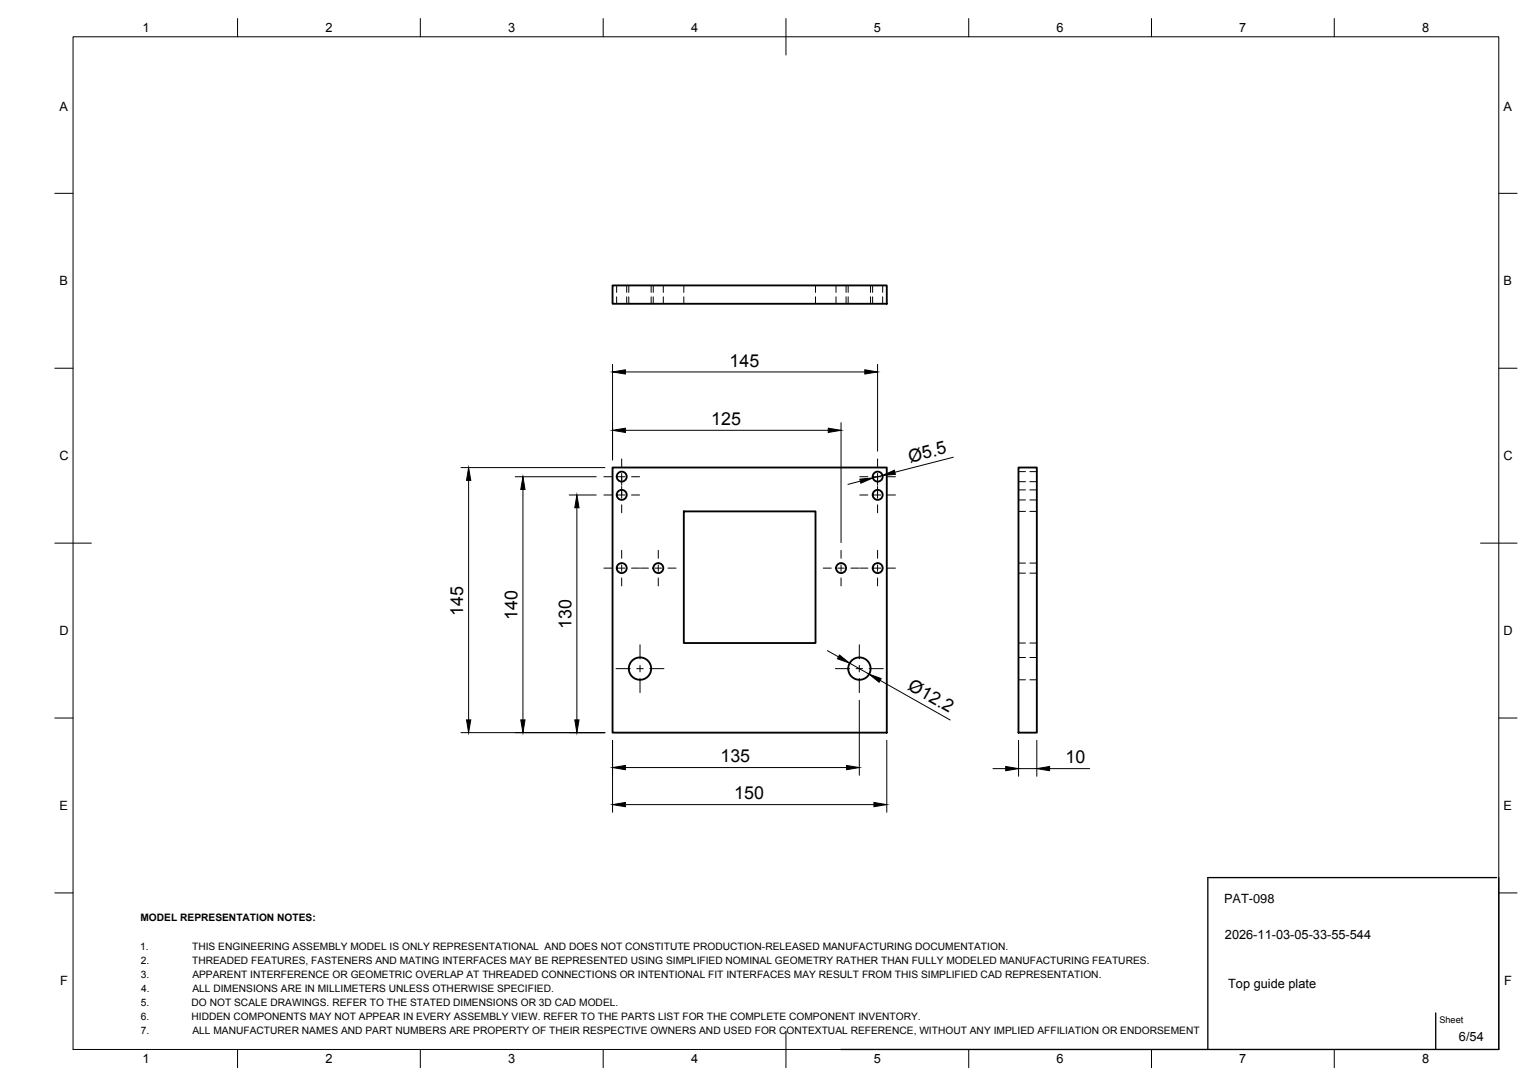
ISO-10303-21;
HEADER;
/* Generated by software containing ST-Developer
 * from STEP Tools, Inc. (www.steptools.com) 
 */

FILE_DESCRIPTION(
/* description */ ('Spring compression tester'),
/* implementation_level */ '2;1');

FILE_NAME(
/* name */ 'Top guide plate.step',
/* time_stamp */ '2026-10-28T03:24:11-07:00',
/* author */ (''),
/* organization */ (''),
/* preprocessor_version */ 'ST-DEVELOPER v20.2',
/* originating_system */ 'Autodesk Translation Framework v15.17.0.0',
/* authorisation */ '');

FILE_SCHEMA (('AUTOMOTIVE_DESIGN { 1 0 10303 214 3 1 1 }'));
ENDSEC;

DATA;
#10=MECHANICAL_DESIGN_GEOMETRIC_PRESENTATION_REPRESENTATION('',(#1107),#43521);
#987=SHAPE_REPRESENTATION_RELATIONSHIP('SRR','None',#43799,#1047);
#1047=ADVANCED_BREP_SHAPE_REPRESENTATION('',(#1182),#43459);
#1107=STYLED_ITEM('',(#44195),#1182);
#1182=MANIFOLD_SOLID_BREP('Body1',#18544);
#1283=FACE_BOUND('',#3318,.T.);
#1284=FACE_BOUND('',#3319,.T.);
#1285=FACE_BOUND('',#3320,.T.);
#1286=FACE_BOUND('',#3321,.T.);
#1287=FACE_BOUND('',#3322,.T.);
#1288=FACE_BOUND('',#3323,.T.);
#1289=FACE_BOUND('',#3324,.T.);
#1290=FACE_BOUND('',#3325,.T.);
#1291=FACE_BOUND('',#3326,.T.);
#1292=FACE_BOUND('',#3327,.T.);
#1293=FACE_BOUND('',#3328,.T.);
#1294=FACE_BOUND('',#3330,.T.);
#1295=FACE_BOUND('',#3331,.T.);
#1296=FACE_BOUND('',#3332,.T.);
#1297=FACE_BOUND('',#3333,.T.);
#1298=FACE_BOUND('',#3334,.T.);
#1299=FACE_BOUND('',#3335,.T.);
#1300=FACE_BOUND('',#3336,.T.);
#1301=FACE_BOUND('',#3337,.T.);
#1302=FACE_BOUND('',#3338,.T.);
#1303=FACE_BOUND('',#3339,.T.);
#1304=FACE_BOUND('',#3340,.T.);
#1615=PLANE('',#19400);
#1616=PLANE('',#19401);
#1617=PLANE('',#19402);
#1618=PLANE('',#19403);
#1619=PLANE('',#19410);
#1620=PLANE('',#19411);
#1621=PLANE('',#19412);
#1622=PLANE('',#19413);
#1623=PLANE('',#19414);
#1624=PLANE('',#19415);
#2216=FACE_OUTER_BOUND('',#3299,.T.);
#2217=FACE_OUTER_BOUND('',#3300,.T.);
#2218=FACE_OUTER_BOUND('',#3301,.T.);
#2219=FACE_OUTER_BOUND('',#3302,.T.);
#2220=FACE_OUTER_BOUND('',#3303,.T.);
#2221=FACE_OUTER_BOUND('',#3304,.T.);
#2222=FACE_OUTER_BOUND('',#3305,.T.);
#2223=FACE_OUTER_BOUND('',#3306,.T.);
#2224=FACE_OUTER_BOUND('',#3307,.T.);
#2225=FACE_OUTER_BOUND('',#3308,.T.);
#2226=FACE_OUTER_BOUND('',#3309,.T.);
#2227=FACE_OUTER_BOUND('',#3310,.T.);
#2228=FACE_OUTER_BOUND('',#3311,.T.);
#2229=FACE_OUTER_BOUND('',#3312,.T.);
#2230=FACE_OUTER_BOUND('',#3313,.T.);
#2231=FACE_OUTER_BOUND('',#3314,.T.);
#2232=FACE_OUTER_BOUND('',#3315,.T.);
#2233=FACE_OUTER_BOUND('',#3316,.T.);
#2234=FACE_OUTER_BOUND('',#3317,.T.);
#2235=FACE_OUTER_BOUND('',#3329,.T.);
#3299=EDGE_LOOP('',(#12433,#12434,#12435,#12436));
#3300=EDGE_LOOP('',(#12437,#12438,#12439,#12440));
#3301=EDGE_LOOP('',(#12441,#12442,#12443,#12444));
#3302=EDGE_LOOP('',(#12445,#12446,#12447,#12448));
#3303=EDGE_LOOP('',(#12449,#12450,#12451,#12452));
#3304=EDGE_LOOP('',(#12453,#12454,#12455,#12456));
#3305=EDGE_LOOP('',(#12457,#12458,#12459,#12460));
#3306=EDGE_LOOP('',(#12461,#12462,#12463,#12464));
#3307=EDGE_LOOP('',(#12465,#12466,#12467,#12468));
#3308=EDGE_LOOP('',(#12469,#12470,#12471,#12472));
#3309=EDGE_LOOP('',(#12473,#12474,#12475,#12476));
#3310=EDGE_LOOP('',(#12477,#12478,#12479,#12480));
#3311=EDGE_LOOP('',(#12481,#12482,#12483,#12484));
#3312=EDGE_LOOP('',(#12485,#12486,#12487,#12488));
#3313=EDGE_LOOP('',(#12489,#12490,#12491,#12492));
#3314=EDGE_LOOP('',(#12493,#12494,#12495,#12496));
#3315=EDGE_LOOP('',(#12497,#12498,#12499,#12500));
#3316=EDGE_LOOP('',(#12501,#12502,#12503,#12504));
#3317=EDGE_LOOP('',(#12505,#12506,#12507,#12508));
#3318=EDGE_LOOP('',(#12509));
#3319=EDGE_LOOP('',(#12510));
#3320=EDGE_LOOP('',(#12511));
#3321=EDGE_LOOP('',(#12512));
#3322=EDGE_LOOP('',(#12513,#12514,#12515,#12516));
#3323=EDGE_LOOP('',(#12517));
#3324=EDGE_LOOP('',(#12518));
#3325=EDGE_LOOP('',(#12519));
#3326=EDGE_LOOP('',(#12520));
#3327=EDGE_LOOP('',(#12521));
#3328=EDGE_LOOP('',(#12522));
#3329=EDGE_LOOP('',(#12523,#12524,#12525,#12526));
#3330=EDGE_LOOP('',(#12527));
#3331=EDGE_LOOP('',(#12528));
#3332=EDGE_LOOP('',(#12529));
#3333=EDGE_LOOP('',(#12530));
#3334=EDGE_LOOP('',(#12531,#12532,#12533,#12534));
#3335=EDGE_LOOP('',(#12535));
#3336=EDGE_LOOP('',(#12536));
#3337=EDGE_LOOP('',(#12537));
#3338=EDGE_LOOP('',(#12538));
#3339=EDGE_LOOP('',(#12539));
#3340=EDGE_LOOP('',(#12540));
#4674=LINE('',#26688,#6106);
#4675=LINE('',#26694,#6107);
#4676=LINE('',#26700,#6108);
#4677=LINE('',#26706,#6109);
#4678=LINE('',#26712,#6110);
#4679=LINE('',#26718,#6111);
#4680=LINE('',#26724,#6112);
#4681=LINE('',#26730,#6113);
#4682=LINE('',#26735,#6114);
#4683=LINE('',#26737,#6115);
#4684=LINE('',#26739,#6116);
#4685=LINE('',#26740,#6117);
#4686=LINE('',#26743,#6118);
#4687=LINE('',#26745,#6119);
#4688=LINE('',#26746,#6120);
#4689=LINE('',#26749,#6121);
#4690=LINE('',#26751,#6122);
#4691=LINE('',#26752,#6123);
#4692=LINE('',#26754,#6124);
#4693=LINE('',#26755,#6125);
#4694=LINE('',#26760,#6126);
#4695=LINE('',#26766,#6127);
#4696=LINE('',#26771,#6128);
#4697=LINE('',#26773,#6129);
#4698=LINE('',#26775,#6130);
#4699=LINE('',#26776,#6131);
#4700=LINE('',#26779,#6132);
#4701=LINE('',#26781,#6133);
#4702=LINE('',#26782,#6134);
#4703=LINE('',#26785,#6135);
#4704=LINE('',#26787,#6136);
#4705=LINE('',#26788,#6137);
#4706=LINE('',#26790,#6138);
#4707=LINE('',#26791,#6139);
#6106=VECTOR('',#21452,0.275);
#6107=VECTOR('',#21459,0.275);
#6108=VECTOR('',#21466,0.275);
#6109=VECTOR('',#21473,0.275);
#6110=VECTOR('',#21480,0.275);
#6111=VECTOR('',#21487,0.275);
#6112=VECTOR('',#21494,0.275);
#6113=VECTOR('',#21501,0.275);
#6114=VECTOR('',#21506,1.);
#6115=VECTOR('',#21507,1.);
#6116=VECTOR('',#21508,1.);
#6117=VECTOR('',#21509,1.);
#6118=VECTOR('',#21512,1.);
#6119=VECTOR('',#21513,1.);
#6120=VECTOR('',#21514,1.);
#6121=VECTOR('',#21517,1.);
#6122=VECTOR('',#21518,1.);
#6123=VECTOR('',#21519,1.);
#6124=VECTOR('',#21522,1.);
#6125=VECTOR('',#21523,1.);
#6126=VECTOR('',#21528,0.61);
#6127=VECTOR('',#21535,0.61);
#6128=VECTOR('',#21540,1.);
#6129=VECTOR('',#21541,1.);
#6130=VECTOR('',#21542,1.);
#6131=VECTOR('',#21543,1.);
#6132=VECTOR('',#21546,1.);
#6133=VECTOR('',#21547,1.);
#6134=VECTOR('',#21548,1.);
#6135=VECTOR('',#21551,1.);
#6136=VECTOR('',#21552,1.);
#6137=VECTOR('',#21553,1.);
#6138=VECTOR('',#21556,1.);
#6139=VECTOR('',#21557,1.);
#7510=CIRCLE('',#19377,0.275);
#7511=CIRCLE('',#19378,0.275);
#7512=CIRCLE('',#19380,0.275);
#7513=CIRCLE('',#19381,0.275);
#7514=CIRCLE('',#19383,0.275);
#7515=CIRCLE('',#19384,0.275);
#7516=CIRCLE('',#19386,0.275);
#7517=CIRCLE('',#19387,0.275);
#7518=CIRCLE('',#19389,0.275);
#7519=CIRCLE('',#19390,0.275);
#7520=CIRCLE('',#19392,0.275);
#7521=CIRCLE('',#19393,0.275);
#7522=CIRCLE('',#19395,0.275);
#7523=CIRCLE('',#19396,0.275);
#7524=CIRCLE('',#19398,0.275);
#7525=CIRCLE('',#19399,0.275);
#7526=CIRCLE('',#19405,0.61);
#7527=CIRCLE('',#19406,0.61);
#7528=CIRCLE('',#19408,0.61);
#7529=CIRCLE('',#19409,0.61);
#8208=VERTEX_POINT('',#26685);
#8209=VERTEX_POINT('',#26687);
#8210=VERTEX_POINT('',#26691);
#8211=VERTEX_POINT('',#26693);
#8212=VERTEX_POINT('',#26697);
#8213=VERTEX_POINT('',#26699);
#8214=VERTEX_POINT('',#26703);
#8215=VERTEX_POINT('',#26705);
#8216=VERTEX_POINT('',#26709);
#8217=VERTEX_POINT('',#26711);
#8218=VERTEX_POINT('',#26715);
#8219=VERTEX_POINT('',#26717);
#8220=VERTEX_POINT('',#26721);
#8221=VERTEX_POINT('',#26723);
#8222=VERTEX_POINT('',#26727);
#8223=VERTEX_POINT('',#26729);
#8224=VERTEX_POINT('',#26733);
#8225=VERTEX_POINT('',#26734);
#8226=VERTEX_POINT('',#26736);
#8227=VERTEX_POINT('',#26738);
#8228=VERTEX_POINT('',#26742);
#8229=VERTEX_POINT('',#26744);
#8230=VERTEX_POINT('',#26748);
#8231=VERTEX_POINT('',#26750);
#8232=VERTEX_POINT('',#26757);
#8233=VERTEX_POINT('',#26759);
#8234=VERTEX_POINT('',#26763);
#8235=VERTEX_POINT('',#26765);
#8236=VERTEX_POINT('',#26769);
#8237=VERTEX_POINT('',#26770);
#8238=VERTEX_POINT('',#26772);
#8239=VERTEX_POINT('',#26774);
#8240=VERTEX_POINT('',#26778);
#8241=VERTEX_POINT('',#26780);
#8242=VERTEX_POINT('',#26784);
#8243=VERTEX_POINT('',#26786);
#9881=EDGE_CURVE('',#8208,#8208,#7510,.T.);
#9882=EDGE_CURVE('',#8208,#8209,#4674,.T.);
#9883=EDGE_CURVE('',#8209,#8209,#7511,.T.);
#9884=EDGE_CURVE('',#8210,#8210,#7512,.T.);
#9885=EDGE_CURVE('',#8210,#8211,#4675,.T.);
#9886=EDGE_CURVE('',#8211,#8211,#7513,.T.);
#9887=EDGE_CURVE('',#8212,#8212,#7514,.T.);
#9888=EDGE_CURVE('',#8212,#8213,#4676,.T.);
#9889=EDGE_CURVE('',#8213,#8213,#7515,.T.);
#9890=EDGE_CURVE('',#8214,#8214,#7516,.T.);
#9891=EDGE_CURVE('',#8214,#8215,#4677,.T.);
#9892=EDGE_CURVE('',#8215,#8215,#7517,.T.);
#9893=EDGE_CURVE('',#8216,#8216,#7518,.T.);
#9894=EDGE_CURVE('',#8216,#8217,#4678,.T.);
#9895=EDGE_CURVE('',#8217,#8217,#7519,.T.);
#9896=EDGE_CURVE('',#8218,#8218,#7520,.T.);
#9897=EDGE_CURVE('',#8218,#8219,#4679,.T.);
#9898=EDGE_CURVE('',#8219,#8219,#7521,.T.);
#9899=EDGE_CURVE('',#8220,#8220,#7522,.T.);
#9900=EDGE_CURVE('',#8220,#8221,#4680,.T.);
#9901=EDGE_CURVE('',#8221,#8221,#7523,.T.);
#9902=EDGE_CURVE('',#8222,#8222,#7524,.T.);
#9903=EDGE_CURVE('',#8222,#8223,#4681,.T.);
#9904=EDGE_CURVE('',#8223,#8223,#7525,.T.);
#9905=EDGE_CURVE('',#8224,#8225,#4682,.T.);
#9906=EDGE_CURVE('',#8226,#8224,#4683,.T.);
#9907=EDGE_CURVE('',#8227,#8226,#4684,.T.);
#9908=EDGE_CURVE('',#8227,#8225,#4685,.T.);
#9909=EDGE_CURVE('',#8225,#8228,#4686,.T.);
#9910=EDGE_CURVE('',#8229,#8227,#4687,.T.);
#9911=EDGE_CURVE('',#8229,#8228,#4688,.T.);
#9912=EDGE_CURVE('',#8228,#8230,#4689,.T.);
#9913=EDGE_CURVE('',#8231,#8229,#4690,.T.);
#9914=EDGE_CURVE('',#8231,#8230,#4691,.T.);
#9915=EDGE_CURVE('',#8230,#8224,#4692,.T.);
#9916=EDGE_CURVE('',#8226,#8231,#4693,.T.);
#9917=EDGE_CURVE('',#8232,#8232,#7526,.T.);
#9918=EDGE_CURVE('',#8232,#8233,#4694,.T.);
#9919=EDGE_CURVE('',#8233,#8233,#7527,.T.);
#9920=EDGE_CURVE('',#8234,#8234,#7528,.T.);
#9921=EDGE_CURVE('',#8234,#8235,#4695,.T.);
#9922=EDGE_CURVE('',#8235,#8235,#7529,.T.);
#9923=EDGE_CURVE('',#8236,#8237,#4696,.T.);
#9924=EDGE_CURVE('',#8237,#8238,#4697,.T.);
#9925=EDGE_CURVE('',#8239,#8238,#4698,.T.);
#9926=EDGE_CURVE('',#8236,#8239,#4699,.T.);
#9927=EDGE_CURVE('',#8240,#8236,#4700,.T.);
#9928=EDGE_CURVE('',#8241,#8239,#4701,.T.);
#9929=EDGE_CURVE('',#8240,#8241,#4702,.T.);
#9930=EDGE_CURVE('',#8242,#8240,#4703,.T.);
#9931=EDGE_CURVE('',#8243,#8241,#4704,.T.);
#9932=EDGE_CURVE('',#8242,#8243,#4705,.T.);
#9933=EDGE_CURVE('',#8237,#8242,#4706,.T.);
#9934=EDGE_CURVE('',#8238,#8243,#4707,.T.);
#12433=ORIENTED_EDGE('',*,*,#9881,.F.);
#12434=ORIENTED_EDGE('',*,*,#9882,.T.);
#12435=ORIENTED_EDGE('',*,*,#9883,.F.);
#12436=ORIENTED_EDGE('',*,*,#9882,.F.);
#12437=ORIENTED_EDGE('',*,*,#9884,.F.);
#12438=ORIENTED_EDGE('',*,*,#9885,.T.);
#12439=ORIENTED_EDGE('',*,*,#9886,.F.);
#12440=ORIENTED_EDGE('',*,*,#9885,.F.);
#12441=ORIENTED_EDGE('',*,*,#9887,.F.);
#12442=ORIENTED_EDGE('',*,*,#9888,.T.);
#12443=ORIENTED_EDGE('',*,*,#9889,.F.);
#12444=ORIENTED_EDGE('',*,*,#9888,.F.);
#12445=ORIENTED_EDGE('',*,*,#9890,.F.);
#12446=ORIENTED_EDGE('',*,*,#9891,.T.);
#12447=ORIENTED_EDGE('',*,*,#9892,.F.);
#12448=ORIENTED_EDGE('',*,*,#9891,.F.);
#12449=ORIENTED_EDGE('',*,*,#9893,.F.);
#12450=ORIENTED_EDGE('',*,*,#9894,.T.);
#12451=ORIENTED_EDGE('',*,*,#9895,.F.);
#12452=ORIENTED_EDGE('',*,*,#9894,.F.);
#12453=ORIENTED_EDGE('',*,*,#9896,.F.);
#12454=ORIENTED_EDGE('',*,*,#9897,.T.);
#12455=ORIENTED_EDGE('',*,*,#9898,.F.);
#12456=ORIENTED_EDGE('',*,*,#9897,.F.);
#12457=ORIENTED_EDGE('',*,*,#9899,.F.);
#12458=ORIENTED_EDGE('',*,*,#9900,.T.);
#12459=ORIENTED_EDGE('',*,*,#9901,.F.);
#12460=ORIENTED_EDGE('',*,*,#9900,.F.);
#12461=ORIENTED_EDGE('',*,*,#9902,.F.);
#12462=ORIENTED_EDGE('',*,*,#9903,.T.);
#12463=ORIENTED_EDGE('',*,*,#9904,.F.);
#12464=ORIENTED_EDGE('',*,*,#9903,.F.);
#12465=ORIENTED_EDGE('',*,*,#9905,.F.);
#12466=ORIENTED_EDGE('',*,*,#9906,.F.);
#12467=ORIENTED_EDGE('',*,*,#9907,.F.);
#12468=ORIENTED_EDGE('',*,*,#9908,.T.);
#12469=ORIENTED_EDGE('',*,*,#9909,.F.);
#12470=ORIENTED_EDGE('',*,*,#9908,.F.);
#12471=ORIENTED_EDGE('',*,*,#9910,.F.);
#12472=ORIENTED_EDGE('',*,*,#9911,.T.);
#12473=ORIENTED_EDGE('',*,*,#9912,.F.);
#12474=ORIENTED_EDGE('',*,*,#9911,.F.);
#12475=ORIENTED_EDGE('',*,*,#9913,.F.);
#12476=ORIENTED_EDGE('',*,*,#9914,.T.);
#12477=ORIENTED_EDGE('',*,*,#9915,.F.);
#12478=ORIENTED_EDGE('',*,*,#9914,.F.);
#12479=ORIENTED_EDGE('',*,*,#9916,.F.);
#12480=ORIENTED_EDGE('',*,*,#9906,.T.);
#12481=ORIENTED_EDGE('',*,*,#9917,.F.);
#12482=ORIENTED_EDGE('',*,*,#9918,.T.);
#12483=ORIENTED_EDGE('',*,*,#9919,.F.);
#12484=ORIENTED_EDGE('',*,*,#9918,.F.);
#12485=ORIENTED_EDGE('',*,*,#9920,.F.);
#12486=ORIENTED_EDGE('',*,*,#9921,.T.);
#12487=ORIENTED_EDGE('',*,*,#9922,.F.);
#12488=ORIENTED_EDGE('',*,*,#9921,.F.);
#12489=ORIENTED_EDGE('',*,*,#9923,.T.);
#12490=ORIENTED_EDGE('',*,*,#9924,.T.);
#12491=ORIENTED_EDGE('',*,*,#9925,.F.);
#12492=ORIENTED_EDGE('',*,*,#9926,.F.);
#12493=ORIENTED_EDGE('',*,*,#9927,.T.);
#12494=ORIENTED_EDGE('',*,*,#9926,.T.);
#12495=ORIENTED_EDGE('',*,*,#9928,.F.);
#12496=ORIENTED_EDGE('',*,*,#9929,.F.);
#12497=ORIENTED_EDGE('',*,*,#9930,.T.);
#12498=ORIENTED_EDGE('',*,*,#9929,.T.);
#12499=ORIENTED_EDGE('',*,*,#9931,.F.);
#12500=ORIENTED_EDGE('',*,*,#9932,.F.);
#12501=ORIENTED_EDGE('',*,*,#9933,.T.);
#12502=ORIENTED_EDGE('',*,*,#9932,.T.);
#12503=ORIENTED_EDGE('',*,*,#9934,.F.);
#12504=ORIENTED_EDGE('',*,*,#9924,.F.);
#12505=ORIENTED_EDGE('',*,*,#9934,.T.);
#12506=ORIENTED_EDGE('',*,*,#9931,.T.);
#12507=ORIENTED_EDGE('',*,*,#9928,.T.);
#12508=ORIENTED_EDGE('',*,*,#9925,.T.);
#12509=ORIENTED_EDGE('',*,*,#9889,.T.);
#12510=ORIENTED_EDGE('',*,*,#9892,.T.);
#12511=ORIENTED_EDGE('',*,*,#9922,.T.);
#12512=ORIENTED_EDGE('',*,*,#9919,.T.);
#12513=ORIENTED_EDGE('',*,*,#9912,.T.);
#12514=ORIENTED_EDGE('',*,*,#9915,.T.);
#12515=ORIENTED_EDGE('',*,*,#9905,.T.);
#12516=ORIENTED_EDGE('',*,*,#9909,.T.);
#12517=ORIENTED_EDGE('',*,*,#9904,.T.);
#12518=ORIENTED_EDGE('',*,*,#9901,.T.);
#12519=ORIENTED_EDGE('',*,*,#9898,.T.);
#12520=ORIENTED_EDGE('',*,*,#9895,.T.);
#12521=ORIENTED_EDGE('',*,*,#9886,.T.);
#12522=ORIENTED_EDGE('',*,*,#9883,.T.);
#12523=ORIENTED_EDGE('',*,*,#9933,.F.);
#12524=ORIENTED_EDGE('',*,*,#9923,.F.);
#12525=ORIENTED_EDGE('',*,*,#9927,.F.);
#12526=ORIENTED_EDGE('',*,*,#9930,.F.);
#12527=ORIENTED_EDGE('',*,*,#9887,.T.);
#12528=ORIENTED_EDGE('',*,*,#9890,.T.);
#12529=ORIENTED_EDGE('',*,*,#9920,.T.);
#12530=ORIENTED_EDGE('',*,*,#9917,.T.);
#12531=ORIENTED_EDGE('',*,*,#9913,.T.);
#12532=ORIENTED_EDGE('',*,*,#9910,.T.);
#12533=ORIENTED_EDGE('',*,*,#9907,.T.);
#12534=ORIENTED_EDGE('',*,*,#9916,.T.);
#12535=ORIENTED_EDGE('',*,*,#9902,.T.);
#12536=ORIENTED_EDGE('',*,*,#9899,.T.);
#12537=ORIENTED_EDGE('',*,*,#9896,.T.);
#12538=ORIENTED_EDGE('',*,*,#9893,.T.);
#12539=ORIENTED_EDGE('',*,*,#9884,.T.);
#12540=ORIENTED_EDGE('',*,*,#9881,.T.);
#17125=CYLINDRICAL_SURFACE('',#19376,0.275);
#17126=CYLINDRICAL_SURFACE('',#19379,0.275);
#17127=CYLINDRICAL_SURFACE('',#19382,0.275);
#17128=CYLINDRICAL_SURFACE('',#19385,0.275);
#17129=CYLINDRICAL_SURFACE('',#19388,0.275);
#17130=CYLINDRICAL_SURFACE('',#19391,0.275);
#17131=CYLINDRICAL_SURFACE('',#19394,0.275);
#17132=CYLINDRICAL_SURFACE('',#19397,0.275);
#17133=CYLINDRICAL_SURFACE('',#19404,0.61);
#17134=CYLINDRICAL_SURFACE('',#19407,0.61);
#17540=ADVANCED_FACE('',(#2216),#17125,.F.);
#17541=ADVANCED_FACE('',(#2217),#17126,.F.);
#17542=ADVANCED_FACE('',(#2218),#17127,.F.);
#17543=ADVANCED_FACE('',(#2219),#17128,.F.);
#17544=ADVANCED_FACE('',(#2220),#17129,.F.);
#17545=ADVANCED_FACE('',(#2221),#17130,.F.);
#17546=ADVANCED_FACE('',(#2222),#17131,.F.);
#17547=ADVANCED_FACE('',(#2223),#17132,.F.);
#17548=ADVANCED_FACE('',(#2224),#1615,.F.);
#17549=ADVANCED_FACE('',(#2225),#1616,.F.);
#17550=ADVANCED_FACE('',(#2226),#1617,.F.);
#17551=ADVANCED_FACE('',(#2227),#1618,.F.);
#17552=ADVANCED_FACE('',(#2228),#17133,.F.);
#17553=ADVANCED_FACE('',(#2229),#17134,.F.);
#17554=ADVANCED_FACE('',(#2230),#1619,.T.);
#17555=ADVANCED_FACE('',(#2231),#1620,.T.);
#17556=ADVANCED_FACE('',(#2232),#1621,.T.);
#17557=ADVANCED_FACE('',(#2233),#1622,.T.);
#17558=ADVANCED_FACE('',(#2234,#1283,#1284,#1285,#1286,#1287,#1288,#1289,
#1290,#1291,#1292,#1293),#1623,.T.);
#17559=ADVANCED_FACE('',(#2235,#1294,#1295,#1296,#1297,#1298,#1299,#1300,
#1301,#1302,#1303,#1304),#1624,.F.);
#18544=CLOSED_SHELL('',(#17540,#17541,#17542,#17543,#17544,#17545,#17546,
#17547,#17548,#17549,#17550,#17551,#17552,#17553,#17554,#17555,#17556,#17557,
#17558,#17559));
#19375=AXIS2_PLACEMENT_3D('',#26683,#21446,#21447);
#19376=AXIS2_PLACEMENT_3D('',#26684,#21448,#21449);
#19377=AXIS2_PLACEMENT_3D('',#26686,#21450,#21451);
#19378=AXIS2_PLACEMENT_3D('',#26689,#21453,#21454);
#19379=AXIS2_PLACEMENT_3D('',#26690,#21455,#21456);
#19380=AXIS2_PLACEMENT_3D('',#26692,#21457,#21458);
#19381=AXIS2_PLACEMENT_3D('',#26695,#21460,#21461);
#19382=AXIS2_PLACEMENT_3D('',#26696,#21462,#21463);
#19383=AXIS2_PLACEMENT_3D('',#26698,#21464,#21465);
#19384=AXIS2_PLACEMENT_3D('',#26701,#21467,#21468);
#19385=AXIS2_PLACEMENT_3D('',#26702,#21469,#21470);
#19386=AXIS2_PLACEMENT_3D('',#26704,#21471,#21472);
#19387=AXIS2_PLACEMENT_3D('',#26707,#21474,#21475);
#19388=AXIS2_PLACEMENT_3D('',#26708,#21476,#21477);
#19389=AXIS2_PLACEMENT_3D('',#26710,#21478,#21479);
#19390=AXIS2_PLACEMENT_3D('',#26713,#21481,#21482);
#19391=AXIS2_PLACEMENT_3D('',#26714,#21483,#21484);
#19392=AXIS2_PLACEMENT_3D('',#26716,#21485,#21486);
#19393=AXIS2_PLACEMENT_3D('',#26719,#21488,#21489);
#19394=AXIS2_PLACEMENT_3D('',#26720,#21490,#21491);
#19395=AXIS2_PLACEMENT_3D('',#26722,#21492,#21493);
#19396=AXIS2_PLACEMENT_3D('',#26725,#21495,#21496);
#19397=AXIS2_PLACEMENT_3D('',#26726,#21497,#21498);
#19398=AXIS2_PLACEMENT_3D('',#26728,#21499,#21500);
#19399=AXIS2_PLACEMENT_3D('',#26731,#21502,#21503);
#19400=AXIS2_PLACEMENT_3D('',#26732,#21504,#21505);
#19401=AXIS2_PLACEMENT_3D('',#26741,#21510,#21511);
#19402=AXIS2_PLACEMENT_3D('',#26747,#21515,#21516);
#19403=AXIS2_PLACEMENT_3D('',#26753,#21520,#21521);
#19404=AXIS2_PLACEMENT_3D('',#26756,#21524,#21525);
#19405=AXIS2_PLACEMENT_3D('',#26758,#21526,#21527);
#19406=AXIS2_PLACEMENT_3D('',#26761,#21529,#21530);
#19407=AXIS2_PLACEMENT_3D('',#26762,#21531,#21532);
#19408=AXIS2_PLACEMENT_3D('',#26764,#21533,#21534);
#19409=AXIS2_PLACEMENT_3D('',#26767,#21536,#21537);
#19410=AXIS2_PLACEMENT_3D('',#26768,#21538,#21539);
#19411=AXIS2_PLACEMENT_3D('',#26777,#21544,#21545);
#19412=AXIS2_PLACEMENT_3D('',#26783,#21549,#21550);
#19413=AXIS2_PLACEMENT_3D('',#26789,#21554,#21555);
#19414=AXIS2_PLACEMENT_3D('',#26792,#21558,#21559);
#19415=AXIS2_PLACEMENT_3D('',#26793,#21560,#21561);
#21446=DIRECTION('axis',(0.,0.,1.));
#21447=DIRECTION('refdir',(1.,0.,0.));
#21448=DIRECTION('center_axis',(0.,0.,1.));
#21449=DIRECTION('ref_axis',(1.,0.,0.));
#21450=DIRECTION('center_axis',(0.,0.,1.));
#21451=DIRECTION('ref_axis',(1.,0.,0.));
#21452=DIRECTION('',(0.,0.,1.));
#21453=DIRECTION('center_axis',(0.,0.,-1.));
#21454=DIRECTION('ref_axis',(1.,0.,0.));
#21455=DIRECTION('center_axis',(0.,0.,1.));
#21456=DIRECTION('ref_axis',(1.,0.,0.));
#21457=DIRECTION('center_axis',(0.,0.,1.));
#21458=DIRECTION('ref_axis',(1.,0.,0.));
#21459=DIRECTION('',(0.,0.,1.));
#21460=DIRECTION('center_axis',(0.,0.,-1.));
#21461=DIRECTION('ref_axis',(1.,0.,0.));
#21462=DIRECTION('center_axis',(0.,0.,1.));
#21463=DIRECTION('ref_axis',(1.,0.,0.));
#21464=DIRECTION('center_axis',(0.,0.,1.));
#21465=DIRECTION('ref_axis',(1.,0.,0.));
#21466=DIRECTION('',(0.,0.,1.));
#21467=DIRECTION('center_axis',(0.,0.,-1.));
#21468=DIRECTION('ref_axis',(1.,0.,0.));
#21469=DIRECTION('center_axis',(0.,0.,1.));
#21470=DIRECTION('ref_axis',(1.,0.,0.));
#21471=DIRECTION('center_axis',(0.,0.,1.));
#21472=DIRECTION('ref_axis',(1.,0.,0.));
#21473=DIRECTION('',(0.,0.,1.));
#21474=DIRECTION('center_axis',(0.,0.,-1.));
#21475=DIRECTION('ref_axis',(1.,0.,0.));
#21476=DIRECTION('center_axis',(0.,0.,1.));
#21477=DIRECTION('ref_axis',(1.,0.,0.));
#21478=DIRECTION('center_axis',(0.,0.,1.));
#21479=DIRECTION('ref_axis',(1.,0.,0.));
#21480=DIRECTION('',(0.,0.,1.));
#21481=DIRECTION('center_axis',(0.,0.,-1.));
#21482=DIRECTION('ref_axis',(1.,0.,0.));
#21483=DIRECTION('center_axis',(0.,0.,1.));
#21484=DIRECTION('ref_axis',(1.,0.,0.));
#21485=DIRECTION('center_axis',(0.,0.,1.));
#21486=DIRECTION('ref_axis',(1.,0.,0.));
#21487=DIRECTION('',(0.,0.,1.));
#21488=DIRECTION('center_axis',(0.,0.,-1.));
#21489=DIRECTION('ref_axis',(1.,0.,0.));
#21490=DIRECTION('center_axis',(0.,0.,1.));
#21491=DIRECTION('ref_axis',(1.,0.,0.));
#21492=DIRECTION('center_axis',(0.,0.,1.));
#21493=DIRECTION('ref_axis',(1.,0.,0.));
#21494=DIRECTION('',(0.,0.,1.));
#21495=DIRECTION('center_axis',(0.,0.,-1.));
#21496=DIRECTION('ref_axis',(1.,0.,0.));
#21497=DIRECTION('center_axis',(0.,0.,1.));
#21498=DIRECTION('ref_axis',(1.,0.,0.));
#21499=DIRECTION('center_axis',(0.,0.,1.));
#21500=DIRECTION('ref_axis',(1.,0.,0.));
#21501=DIRECTION('',(0.,0.,1.));
#21502=DIRECTION('center_axis',(0.,0.,-1.));
#21503=DIRECTION('ref_axis',(1.,0.,0.));
#21504=DIRECTION('center_axis',(0.,-1.,0.));
#21505=DIRECTION('ref_axis',(1.,0.,0.));
#21506=DIRECTION('',(-1.,0.,0.));
#21507=DIRECTION('',(0.,0.,1.));
#21508=DIRECTION('',(1.,0.,0.));
#21509=DIRECTION('',(0.,0.,1.));
#21510=DIRECTION('center_axis',(-1.,0.,0.));
#21511=DIRECTION('ref_axis',(0.,-1.,0.));
#21512=DIRECTION('',(0.,1.,0.));
#21513=DIRECTION('',(0.,-1.,0.));
#21514=DIRECTION('',(0.,0.,1.));
#21515=DIRECTION('center_axis',(0.,1.,0.));
#21516=DIRECTION('ref_axis',(-1.,0.,0.));
#21517=DIRECTION('',(1.,0.,0.));
#21518=DIRECTION('',(-1.,0.,0.));
#21519=DIRECTION('',(0.,0.,1.));
#21520=DIRECTION('center_axis',(1.,0.,0.));
#21521=DIRECTION('ref_axis',(0.,1.,0.));
#21522=DIRECTION('',(0.,-1.,0.));
#21523=DIRECTION('',(0.,1.,0.));
#21524=DIRECTION('center_axis',(0.,0.,1.));
#21525=DIRECTION('ref_axis',(1.,0.,0.));
#21526=DIRECTION('center_axis',(0.,0.,1.));
#21527=DIRECTION('ref_axis',(1.,0.,0.));
#21528=DIRECTION('',(0.,0.,1.));
#21529=DIRECTION('center_axis',(0.,0.,-1.));
#21530=DIRECTION('ref_axis',(1.,0.,0.));
#21531=DIRECTION('center_axis',(0.,0.,1.));
#21532=DIRECTION('ref_axis',(1.,0.,0.));
#21533=DIRECTION('center_axis',(0.,0.,1.));
#21534=DIRECTION('ref_axis',(1.,0.,0.));
#21535=DIRECTION('',(0.,0.,1.));
#21536=DIRECTION('center_axis',(0.,0.,-1.));
#21537=DIRECTION('ref_axis',(1.,0.,0.));
#21538=DIRECTION('center_axis',(0.,1.,0.));
#21539=DIRECTION('ref_axis',(-1.,0.,0.));
#21540=DIRECTION('',(-1.,0.,0.));
#21541=DIRECTION('',(0.,0.,1.));
#21542=DIRECTION('',(-1.,0.,0.));
#21543=DIRECTION('',(0.,0.,1.));
#21544=DIRECTION('center_axis',(1.,0.,0.));
#21545=DIRECTION('ref_axis',(0.,1.,0.));
#21546=DIRECTION('',(0.,1.,0.));
#21547=DIRECTION('',(0.,1.,0.));
#21548=DIRECTION('',(0.,0.,1.));
#21549=DIRECTION('center_axis',(0.,-1.,0.));
#21550=DIRECTION('ref_axis',(1.,0.,0.));
#21551=DIRECTION('',(1.,0.,0.));
#21552=DIRECTION('',(1.,0.,0.));
#21553=DIRECTION('',(0.,0.,1.));
#21554=DIRECTION('center_axis',(-1.,0.,0.));
#21555=DIRECTION('ref_axis',(0.,-1.,0.));
#21556=DIRECTION('',(0.,-1.,0.));
#21557=DIRECTION('',(0.,-1.,0.));
#21558=DIRECTION('center_axis',(0.,0.,1.));
#21559=DIRECTION('ref_axis',(1.,0.,0.));
#21560=DIRECTION('center_axis',(0.,0.,1.));
#21561=DIRECTION('ref_axis',(1.,0.,0.));
#26683=CARTESIAN_POINT('',(0.,0.,0.));
#26684=CARTESIAN_POINT('Origin',(5.,5.5,30.4));
#26685=CARTESIAN_POINT('',(4.725,5.5,30.5));
#26686=CARTESIAN_POINT('Origin',(5.,5.5,30.5));
#26687=CARTESIAN_POINT('',(4.725,5.5,31.5));
#26688=CARTESIAN_POINT('',(4.725,5.5,30.4));
#26689=CARTESIAN_POINT('Origin',(5.,5.5,31.5));
#26690=CARTESIAN_POINT('Origin',(7.,5.5,30.4));
#26691=CARTESIAN_POINT('',(6.725,5.5,30.5));
#26692=CARTESIAN_POINT('Origin',(7.,5.5,30.5));
#26693=CARTESIAN_POINT('',(6.725,5.5,31.5));
#26694=CARTESIAN_POINT('',(6.725,5.5,30.4));
#26695=CARTESIAN_POINT('Origin',(7.,5.5,31.5));
#26696=CARTESIAN_POINT('Origin',(-7.,5.5,30.4));
#26697=CARTESIAN_POINT('',(-7.275,5.5,30.5));
#26698=CARTESIAN_POINT('Origin',(-7.,5.5,30.5));
#26699=CARTESIAN_POINT('',(-7.275,5.5,31.5));
#26700=CARTESIAN_POINT('',(-7.275,5.5,30.4));
#26701=CARTESIAN_POINT('Origin',(-7.,5.5,31.5));
#26702=CARTESIAN_POINT('Origin',(-5.,5.5,30.4));
#26703=CARTESIAN_POINT('',(-5.275,5.5,30.5));
#26704=CARTESIAN_POINT('Origin',(-5.,5.5,30.5));
#26705=CARTESIAN_POINT('',(-5.275,5.5,31.5));
#26706=CARTESIAN_POINT('',(-5.275,5.5,30.4));
#26707=CARTESIAN_POINT('Origin',(-5.,5.5,31.5));
#26708=CARTESIAN_POINT('Origin',(7.,9.5,30.4));
#26709=CARTESIAN_POINT('',(6.725,9.5,30.5));
#26710=CARTESIAN_POINT('Origin',(7.,9.5,30.5));
#26711=CARTESIAN_POINT('',(6.725,9.5,31.5));
#26712=CARTESIAN_POINT('',(6.725,9.5,30.4));
#26713=CARTESIAN_POINT('Origin',(7.,9.5,31.5));
#26714=CARTESIAN_POINT('Origin',(7.,10.5,30.4));
#26715=CARTESIAN_POINT('',(6.725,10.5,30.5));
#26716=CARTESIAN_POINT('Origin',(7.,10.5,30.5));
#26717=CARTESIAN_POINT('',(6.725,10.5,31.5));
#26718=CARTESIAN_POINT('',(6.725,10.5,30.4));
#26719=CARTESIAN_POINT('Origin',(7.,10.5,31.5));
#26720=CARTESIAN_POINT('Origin',(-7.,9.5,30.4));
#26721=CARTESIAN_POINT('',(-7.275,9.5,30.5));
#26722=CARTESIAN_POINT('Origin',(-7.,9.5,30.5));
#26723=CARTESIAN_POINT('',(-7.275,9.5,31.5));
#26724=CARTESIAN_POINT('',(-7.275,9.5,30.4));
#26725=CARTESIAN_POINT('Origin',(-7.,9.5,31.5));
#26726=CARTESIAN_POINT('Origin',(-7.,10.5,30.4));
#26727=CARTESIAN_POINT('',(-7.275,10.5,30.5));
#26728=CARTESIAN_POINT('Origin',(-7.,10.5,30.5));
#26729=CARTESIAN_POINT('',(-7.275,10.5,31.5));
#26730=CARTESIAN_POINT('',(-7.275,10.5,30.4));
#26731=CARTESIAN_POINT('Origin',(-7.,10.5,31.5));
#26732=CARTESIAN_POINT('Origin',(-3.6,1.4,30.4));
#26733=CARTESIAN_POINT('',(3.6,1.4,31.5));
#26734=CARTESIAN_POINT('',(-3.6,1.4,31.5));
#26735=CARTESIAN_POINT('',(-1.8,1.4,31.5));
#26736=CARTESIAN_POINT('',(3.6,1.4,30.5));
#26737=CARTESIAN_POINT('',(3.6,1.4,30.4));
#26738=CARTESIAN_POINT('',(-3.6,1.4,30.5));
#26739=CARTESIAN_POINT('',(-1.8,1.4,30.5));
#26740=CARTESIAN_POINT('',(-3.6,1.4,30.4));
#26741=CARTESIAN_POINT('Origin',(-3.6,8.6,30.4));
#26742=CARTESIAN_POINT('',(-3.6,8.6,31.5));
#26743=CARTESIAN_POINT('',(-3.6,6.175,31.5));
#26744=CARTESIAN_POINT('',(-3.6,8.6,30.5));
#26745=CARTESIAN_POINT('',(-3.6,6.175,30.5));
#26746=CARTESIAN_POINT('',(-3.6,8.6,30.4));
#26747=CARTESIAN_POINT('Origin',(3.6,8.6,30.4));
#26748=CARTESIAN_POINT('',(3.6,8.6,31.5));
#26749=CARTESIAN_POINT('',(1.8,8.6,31.5));
#26750=CARTESIAN_POINT('',(3.6,8.6,30.5));
#26751=CARTESIAN_POINT('',(1.8,8.6,30.5));
#26752=CARTESIAN_POINT('',(3.6,8.6,30.4));
#26753=CARTESIAN_POINT('Origin',(3.6,1.4,30.4));
#26754=CARTESIAN_POINT('',(3.6,2.575,31.5));
#26755=CARTESIAN_POINT('',(3.6,2.575,30.5));
#26756=CARTESIAN_POINT('Origin',(-6.,0.,30.4));
#26757=CARTESIAN_POINT('',(-6.61,-7.47034547479886E-17,30.5));
#26758=CARTESIAN_POINT('Origin',(-6.,0.,30.5));
#26759=CARTESIAN_POINT('',(-6.61,7.47034547479886E-17,31.5));
#26760=CARTESIAN_POINT('',(-6.61,-7.47034547479886E-17,30.4));
#26761=CARTESIAN_POINT('Origin',(-6.,0.,31.5));
#26762=CARTESIAN_POINT('Origin',(6.,0.,30.4));
#26763=CARTESIAN_POINT('',(5.39,-7.47034547479886E-17,30.5));
#26764=CARTESIAN_POINT('Origin',(6.,0.,30.5));
#26765=CARTESIAN_POINT('',(5.39,7.47034547479886E-17,31.5));
#26766=CARTESIAN_POINT('',(5.39,-7.47034547479886E-17,30.4));
#26767=CARTESIAN_POINT('Origin',(6.,0.,31.5));
#26768=CARTESIAN_POINT('Origin',(7.5,11.,30.5));
#26769=CARTESIAN_POINT('',(7.5,11.,30.5));
#26770=CARTESIAN_POINT('',(-7.5,11.,30.5));
#26771=CARTESIAN_POINT('',(7.5,11.,30.5));
#26772=CARTESIAN_POINT('',(-7.5,11.,31.5));
#26773=CARTESIAN_POINT('',(-7.5,11.,30.5));
#26774=CARTESIAN_POINT('',(7.5,11.,31.5));
#26775=CARTESIAN_POINT('',(7.5,11.,31.5));
#26776=CARTESIAN_POINT('',(7.5,11.,30.5));
#26777=CARTESIAN_POINT('Origin',(7.5,-3.5,30.5));
#26778=CARTESIAN_POINT('',(7.5,-3.5,30.5));
#26779=CARTESIAN_POINT('',(7.5,-3.5,30.5));
#26780=CARTESIAN_POINT('',(7.5,-3.5,31.5));
#26781=CARTESIAN_POINT('',(7.5,-3.5,31.5));
#26782=CARTESIAN_POINT('',(7.5,-3.5,30.5));
#26783=CARTESIAN_POINT('Origin',(-7.5,-3.5,30.5));
#26784=CARTESIAN_POINT('',(-7.5,-3.5,30.5));
#26785=CARTESIAN_POINT('',(-7.5,-3.5,30.5));
#26786=CARTESIAN_POINT('',(-7.5,-3.5,31.5));
#26787=CARTESIAN_POINT('',(-7.5,-3.5,31.5));
#26788=CARTESIAN_POINT('',(-7.5,-3.5,30.5));
#26789=CARTESIAN_POINT('Origin',(-7.5,11.,30.5));
#26790=CARTESIAN_POINT('',(-7.5,11.,30.5));
#26791=CARTESIAN_POINT('',(-7.5,11.,31.5));
#26792=CARTESIAN_POINT('Origin',(0.,3.75,31.5));
#26793=CARTESIAN_POINT('Origin',(0.,3.75,30.5));
#43391=UNCERTAINTY_MEASURE_WITH_UNIT(LENGTH_MEASURE(0.001),#43522,
'DISTANCE_ACCURACY_VALUE',
'Maximum model space distance between geometric entities at asserted c
onnectivities');
#43453=UNCERTAINTY_MEASURE_WITH_UNIT(LENGTH_MEASURE(0.001),#43522,
'DISTANCE_ACCURACY_VALUE',
'Maximum model space distance between geometric entities at asserted c
onnectivities');
#43459=(
GEOMETRIC_REPRESENTATION_CONTEXT(3)
GLOBAL_UNCERTAINTY_ASSIGNED_CONTEXT((#43391))
GLOBAL_UNIT_ASSIGNED_CONTEXT((#43522,#43524,#43525))
REPRESENTATION_CONTEXT('','3D')
);
#43521=(
GEOMETRIC_REPRESENTATION_CONTEXT(3)
GLOBAL_UNCERTAINTY_ASSIGNED_CONTEXT((#43453))
GLOBAL_UNIT_ASSIGNED_CONTEXT((#43522,#43524,#43525))
REPRESENTATION_CONTEXT('','3D')
);
#43522=(
LENGTH_UNIT()
NAMED_UNIT(*)
SI_UNIT(.CENTI.,.METRE.)
);
#43524=(
NAMED_UNIT(*)
PLANE_ANGLE_UNIT()
SI_UNIT($,.RADIAN.)
);
#43525=(
NAMED_UNIT(*)
SI_UNIT($,.STERADIAN.)
SOLID_ANGLE_UNIT()
);
#43531=SHAPE_DEFINITION_REPRESENTATION(#43598,#43799);
#43598=PRODUCT_DEFINITION_SHAPE('',$,#43867);
#43799=SHAPE_REPRESENTATION('',(#19375),#43459);
#43861=PRODUCT_DEFINITION_CONTEXT('part definition',#44064,'design');
#43867=PRODUCT_DEFINITION('Top guide plate','Top guide plate',#43934,#43861);
#43934=PRODUCT_DEFINITION_FORMATION('',$,#44071);
#44064=APPLICATION_CONTEXT(
'Core Data for Automotive Mechanical Design Process');
#44065=PRODUCT_CONTEXT('part definition',#44064,'mechanical');
#44071=PRODUCT('Top guide plate','Top guide plate','Top guide plate',(#44065));
#44189=COLOUR_RGB('Sky Blue',0.24,0.69,0.87);
#44190=FILL_AREA_STYLE_COLOUR('',#44189);
#44191=FILL_AREA_STYLE('',(#44190));
#44192=SURFACE_STYLE_FILL_AREA(#44191);
#44193=SURFACE_SIDE_STYLE('',(#44192));
#44194=SURFACE_STYLE_USAGE(.BOTH.,#44193);
#44195=PRESENTATION_STYLE_ASSIGNMENT((#44194));
ENDSEC;
END-ISO-10303-21;
